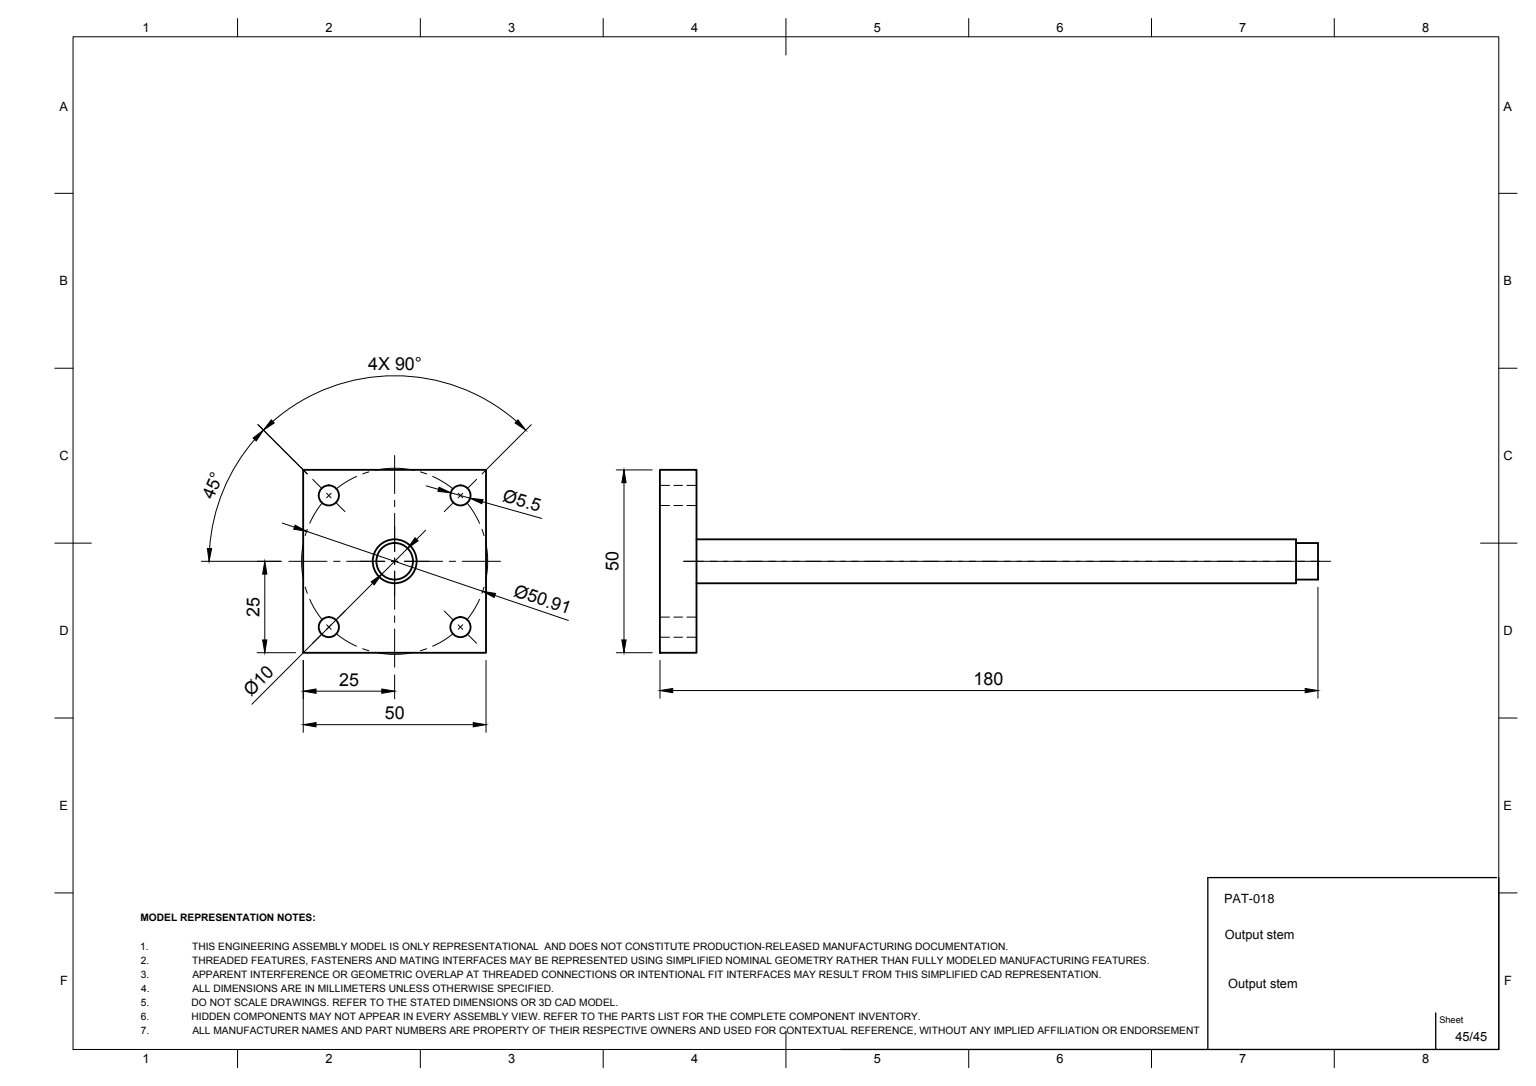
ISO-10303-21;
HEADER;
/* Generated by software containing ST-Developer
 * from STEP Tools, Inc. (www.steptools.com) 
 */

FILE_DESCRIPTION(
/* description */ ('Cam-driven reciprocating slide'),
/* implementation_level */ '2;1');

FILE_NAME(
/* name */ 'Output stem.step',
/* time_stamp */ '2026-10-28T03:25:20-07:00',
/* author */ (''),
/* organization */ (''),
/* preprocessor_version */ 'ST-DEVELOPER v20.2',
/* originating_system */ 'Autodesk Translation Framework v15.17.0.0',
/* authorisation */ '');

FILE_SCHEMA (('AUTOMOTIVE_DESIGN { 1 0 10303 214 3 1 1 }'));
ENDSEC;

DATA;
#10=MECHANICAL_DESIGN_GEOMETRIC_PRESENTATION_REPRESENTATION('',(#464),#13277);
#383=SHAPE_REPRESENTATION_RELATIONSHIP('SRR','None',#13480,#420);
#420=ADVANCED_BREP_SHAPE_REPRESENTATION('',(#505),#13275);
#464=STYLED_ITEM('',(#13706),#505);
#505=MANIFOLD_SOLID_BREP('Body1',#6443);
#669=FACE_BOUND('',#1808,.T.);
#670=FACE_BOUND('',#1809,.T.);
#671=FACE_BOUND('',#1810,.T.);
#672=FACE_BOUND('',#1811,.T.);
#673=FACE_BOUND('',#1812,.T.);
#674=FACE_BOUND('',#1818,.T.);
#675=FACE_BOUND('',#1819,.T.);
#676=FACE_BOUND('',#1820,.T.);
#677=FACE_BOUND('',#1821,.T.);
#678=FACE_BOUND('',#1826,.T.);
#891=PLANE('',#7640);
#892=PLANE('',#7642);
#893=PLANE('',#7643);
#894=PLANE('',#7644);
#895=PLANE('',#7645);
#896=PLANE('',#7646);
#897=PLANE('',#7650);
#898=PLANE('',#7653);
#1262=FACE_OUTER_BOUND('',#1803,.T.);
#1263=FACE_OUTER_BOUND('',#1804,.T.);
#1264=FACE_OUTER_BOUND('',#1805,.T.);
#1265=FACE_OUTER_BOUND('',#1806,.T.);
#1266=FACE_OUTER_BOUND('',#1807,.T.);
#1267=FACE_OUTER_BOUND('',#1813,.T.);
#1268=FACE_OUTER_BOUND('',#1814,.T.);
#1269=FACE_OUTER_BOUND('',#1815,.T.);
#1270=FACE_OUTER_BOUND('',#1816,.T.);
#1271=FACE_OUTER_BOUND('',#1817,.T.);
#1272=FACE_OUTER_BOUND('',#1822,.T.);
#1273=FACE_OUTER_BOUND('',#1823,.T.);
#1274=FACE_OUTER_BOUND('',#1824,.T.);
#1275=FACE_OUTER_BOUND('',#1825,.T.);
#1803=EDGE_LOOP('',(#5820,#5821,#5822,#5823));
#1804=EDGE_LOOP('',(#5824,#5825,#5826,#5827));
#1805=EDGE_LOOP('',(#5828,#5829,#5830,#5831));
#1806=EDGE_LOOP('',(#5832,#5833,#5834,#5835));
#1807=EDGE_LOOP('',(#5836,#5837,#5838,#5839));
#1808=EDGE_LOOP('',(#5840));
#1809=EDGE_LOOP('',(#5841));
#1810=EDGE_LOOP('',(#5842));
#1811=EDGE_LOOP('',(#5843));
#1812=EDGE_LOOP('',(#5844));
#1813=EDGE_LOOP('',(#5845,#5846,#5847,#5848));
#1814=EDGE_LOOP('',(#5849,#5850,#5851,#5852));
#1815=EDGE_LOOP('',(#5853,#5854,#5855,#5856));
#1816=EDGE_LOOP('',(#5857,#5858,#5859,#5860));
#1817=EDGE_LOOP('',(#5861,#5862,#5863,#5864));
#1818=EDGE_LOOP('',(#5865));
#1819=EDGE_LOOP('',(#5866));
#1820=EDGE_LOOP('',(#5867));
#1821=EDGE_LOOP('',(#5868));
#1822=EDGE_LOOP('',(#5869,#5870,#5871,#5872));
#1823=EDGE_LOOP('',(#5873));
#1824=EDGE_LOOP('',(#5874,#5875,#5876,#5877));
#1825=EDGE_LOOP('',(#5878));
#1826=EDGE_LOOP('',(#5879));
#2252=LINE('',#13109,#2691);
#2253=LINE('',#13115,#2692);
#2254=LINE('',#13121,#2693);
#2255=LINE('',#13127,#2694);
#2256=LINE('',#13132,#2695);
#2257=LINE('',#13134,#2696);
#2258=LINE('',#13136,#2697);
#2259=LINE('',#13137,#2698);
#2260=LINE('',#13142,#2699);
#2261=LINE('',#13144,#2700);
#2262=LINE('',#13145,#2701);
#2263=LINE('',#13148,#2702);
#2264=LINE('',#13149,#2703);
#2265=LINE('',#13152,#2704);
#2266=LINE('',#13153,#2705);
#2267=LINE('',#13155,#2706);
#2268=LINE('',#13161,#2707);
#2269=LINE('',#13166,#2708);
#2691=VECTOR('',#9642,0.275);
#2692=VECTOR('',#9649,0.275);
#2693=VECTOR('',#9656,0.275);
#2694=VECTOR('',#9663,0.275);
#2695=VECTOR('',#9668,1.);
#2696=VECTOR('',#9669,1.);
#2697=VECTOR('',#9670,1.);
#2698=VECTOR('',#9671,1.);
#2699=VECTOR('',#9676,1.);
#2700=VECTOR('',#9677,1.);
#2701=VECTOR('',#9678,1.);
#2702=VECTOR('',#9681,1.);
#2703=VECTOR('',#9682,1.);
#2704=VECTOR('',#9685,1.);
#2705=VECTOR('',#9686,1.);
#2706=VECTOR('',#9689,1.);
#2707=VECTOR('',#9696,0.5);
#2708=VECTOR('',#9703,0.6);
#3019=CIRCLE('',#7629,0.275);
#3020=CIRCLE('',#7630,0.275);
#3021=CIRCLE('',#7632,0.275);
#3022=CIRCLE('',#7633,0.275);
#3023=CIRCLE('',#7635,0.275);
#3024=CIRCLE('',#7636,0.275);
#3025=CIRCLE('',#7638,0.275);
#3026=CIRCLE('',#7639,0.275);
#3027=CIRCLE('',#7641,0.6);
#3028=CIRCLE('',#7648,0.5);
#3029=CIRCLE('',#7649,0.5);
#3030=CIRCLE('',#7652,0.6);
#3534=VERTEX_POINT('',#13106);
#3535=VERTEX_POINT('',#13108);
#3536=VERTEX_POINT('',#13112);
#3537=VERTEX_POINT('',#13114);
#3538=VERTEX_POINT('',#13118);
#3539=VERTEX_POINT('',#13120);
#3540=VERTEX_POINT('',#13124);
#3541=VERTEX_POINT('',#13126);
#3542=VERTEX_POINT('',#13130);
#3543=VERTEX_POINT('',#13131);
#3544=VERTEX_POINT('',#13133);
#3545=VERTEX_POINT('',#13135);
#3546=VERTEX_POINT('',#13138);
#3547=VERTEX_POINT('',#13141);
#3548=VERTEX_POINT('',#13143);
#3549=VERTEX_POINT('',#13147);
#3550=VERTEX_POINT('',#13151);
#3551=VERTEX_POINT('',#13158);
#3552=VERTEX_POINT('',#13160);
#3553=VERTEX_POINT('',#13165);
#4300=EDGE_CURVE('',#3534,#3534,#3019,.T.);
#4301=EDGE_CURVE('',#3534,#3535,#2252,.T.);
#4302=EDGE_CURVE('',#3535,#3535,#3020,.T.);
#4303=EDGE_CURVE('',#3536,#3536,#3021,.T.);
#4304=EDGE_CURVE('',#3536,#3537,#2253,.T.);
#4305=EDGE_CURVE('',#3537,#3537,#3022,.T.);
#4306=EDGE_CURVE('',#3538,#3538,#3023,.T.);
#4307=EDGE_CURVE('',#3538,#3539,#2254,.T.);
#4308=EDGE_CURVE('',#3539,#3539,#3024,.T.);
#4309=EDGE_CURVE('',#3540,#3540,#3025,.T.);
#4310=EDGE_CURVE('',#3540,#3541,#2255,.T.);
#4311=EDGE_CURVE('',#3541,#3541,#3026,.T.);
#4312=EDGE_CURVE('',#3542,#3543,#2256,.T.);
#4313=EDGE_CURVE('',#3544,#3542,#2257,.T.);
#4314=EDGE_CURVE('',#3545,#3544,#2258,.T.);
#4315=EDGE_CURVE('',#3543,#3545,#2259,.T.);
#4316=EDGE_CURVE('',#3546,#3546,#3027,.T.);
#4317=EDGE_CURVE('',#3542,#3547,#2260,.T.);
#4318=EDGE_CURVE('',#3548,#3547,#2261,.T.);
#4319=EDGE_CURVE('',#3544,#3548,#2262,.T.);
#4320=EDGE_CURVE('',#3549,#3548,#2263,.T.);
#4321=EDGE_CURVE('',#3545,#3549,#2264,.T.);
#4322=EDGE_CURVE('',#3550,#3549,#2265,.T.);
#4323=EDGE_CURVE('',#3543,#3550,#2266,.T.);
#4324=EDGE_CURVE('',#3547,#3550,#2267,.T.);
#4325=EDGE_CURVE('',#3551,#3551,#3028,.T.);
#4326=EDGE_CURVE('',#3551,#3552,#2268,.T.);
#4327=EDGE_CURVE('',#3552,#3552,#3029,.T.);
#4328=EDGE_CURVE('',#3546,#3553,#2269,.T.);
#4329=EDGE_CURVE('',#3553,#3553,#3030,.T.);
#5820=ORIENTED_EDGE('',*,*,#4300,.F.);
#5821=ORIENTED_EDGE('',*,*,#4301,.T.);
#5822=ORIENTED_EDGE('',*,*,#4302,.F.);
#5823=ORIENTED_EDGE('',*,*,#4301,.F.);
#5824=ORIENTED_EDGE('',*,*,#4303,.F.);
#5825=ORIENTED_EDGE('',*,*,#4304,.T.);
#5826=ORIENTED_EDGE('',*,*,#4305,.F.);
#5827=ORIENTED_EDGE('',*,*,#4304,.F.);
#5828=ORIENTED_EDGE('',*,*,#4306,.F.);
#5829=ORIENTED_EDGE('',*,*,#4307,.T.);
#5830=ORIENTED_EDGE('',*,*,#4308,.F.);
#5831=ORIENTED_EDGE('',*,*,#4307,.F.);
#5832=ORIENTED_EDGE('',*,*,#4309,.F.);
#5833=ORIENTED_EDGE('',*,*,#4310,.T.);
#5834=ORIENTED_EDGE('',*,*,#4311,.F.);
#5835=ORIENTED_EDGE('',*,*,#4310,.F.);
#5836=ORIENTED_EDGE('',*,*,#4312,.F.);
#5837=ORIENTED_EDGE('',*,*,#4313,.F.);
#5838=ORIENTED_EDGE('',*,*,#4314,.F.);
#5839=ORIENTED_EDGE('',*,*,#4315,.F.);
#5840=ORIENTED_EDGE('',*,*,#4316,.T.);
#5841=ORIENTED_EDGE('',*,*,#4309,.T.);
#5842=ORIENTED_EDGE('',*,*,#4306,.T.);
#5843=ORIENTED_EDGE('',*,*,#4303,.T.);
#5844=ORIENTED_EDGE('',*,*,#4300,.T.);
#5845=ORIENTED_EDGE('',*,*,#4313,.T.);
#5846=ORIENTED_EDGE('',*,*,#4317,.T.);
#5847=ORIENTED_EDGE('',*,*,#4318,.F.);
#5848=ORIENTED_EDGE('',*,*,#4319,.F.);
#5849=ORIENTED_EDGE('',*,*,#4314,.T.);
#5850=ORIENTED_EDGE('',*,*,#4319,.T.);
#5851=ORIENTED_EDGE('',*,*,#4320,.F.);
#5852=ORIENTED_EDGE('',*,*,#4321,.F.);
#5853=ORIENTED_EDGE('',*,*,#4315,.T.);
#5854=ORIENTED_EDGE('',*,*,#4321,.T.);
#5855=ORIENTED_EDGE('',*,*,#4322,.F.);
#5856=ORIENTED_EDGE('',*,*,#4323,.F.);
#5857=ORIENTED_EDGE('',*,*,#4312,.T.);
#5858=ORIENTED_EDGE('',*,*,#4323,.T.);
#5859=ORIENTED_EDGE('',*,*,#4324,.F.);
#5860=ORIENTED_EDGE('',*,*,#4317,.F.);
#5861=ORIENTED_EDGE('',*,*,#4324,.T.);
#5862=ORIENTED_EDGE('',*,*,#4322,.T.);
#5863=ORIENTED_EDGE('',*,*,#4320,.T.);
#5864=ORIENTED_EDGE('',*,*,#4318,.T.);
#5865=ORIENTED_EDGE('',*,*,#4302,.T.);
#5866=ORIENTED_EDGE('',*,*,#4305,.T.);
#5867=ORIENTED_EDGE('',*,*,#4308,.T.);
#5868=ORIENTED_EDGE('',*,*,#4311,.T.);
#5869=ORIENTED_EDGE('',*,*,#4325,.F.);
#5870=ORIENTED_EDGE('',*,*,#4326,.T.);
#5871=ORIENTED_EDGE('',*,*,#4327,.T.);
#5872=ORIENTED_EDGE('',*,*,#4326,.F.);
#5873=ORIENTED_EDGE('',*,*,#4327,.F.);
#5874=ORIENTED_EDGE('',*,*,#4316,.F.);
#5875=ORIENTED_EDGE('',*,*,#4328,.T.);
#5876=ORIENTED_EDGE('',*,*,#4329,.T.);
#5877=ORIENTED_EDGE('',*,*,#4328,.F.);
#5878=ORIENTED_EDGE('',*,*,#4329,.F.);
#5879=ORIENTED_EDGE('',*,*,#4325,.T.);
#6011=CYLINDRICAL_SURFACE('',#7628,0.275);
#6012=CYLINDRICAL_SURFACE('',#7631,0.275);
#6013=CYLINDRICAL_SURFACE('',#7634,0.275);
#6014=CYLINDRICAL_SURFACE('',#7637,0.275);
#6015=CYLINDRICAL_SURFACE('',#7647,0.5);
#6016=CYLINDRICAL_SURFACE('',#7651,0.6);
#6380=ADVANCED_FACE('',(#1262),#6011,.F.);
#6381=ADVANCED_FACE('',(#1263),#6012,.F.);
#6382=ADVANCED_FACE('',(#1264),#6013,.F.);
#6383=ADVANCED_FACE('',(#1265),#6014,.F.);
#6384=ADVANCED_FACE('',(#1266,#669,#670,#671,#672,#673),#891,.F.);
#6385=ADVANCED_FACE('',(#1267),#892,.T.);
#6386=ADVANCED_FACE('',(#1268),#893,.T.);
#6387=ADVANCED_FACE('',(#1269),#894,.T.);
#6388=ADVANCED_FACE('',(#1270),#895,.T.);
#6389=ADVANCED_FACE('',(#1271,#674,#675,#676,#677),#896,.T.);
#6390=ADVANCED_FACE('',(#1272),#6015,.T.);
#6391=ADVANCED_FACE('',(#1273),#897,.F.);
#6392=ADVANCED_FACE('',(#1274),#6016,.T.);
#6393=ADVANCED_FACE('',(#1275,#678),#898,.F.);
#6443=CLOSED_SHELL('',(#6380,#6381,#6382,#6383,#6384,#6385,#6386,#6387,
#6388,#6389,#6390,#6391,#6392,#6393));
#7627=AXIS2_PLACEMENT_3D('',#13104,#9636,#9637);
#7628=AXIS2_PLACEMENT_3D('',#13105,#9638,#9639);
#7629=AXIS2_PLACEMENT_3D('',#13107,#9640,#9641);
#7630=AXIS2_PLACEMENT_3D('',#13110,#9643,#9644);
#7631=AXIS2_PLACEMENT_3D('',#13111,#9645,#9646);
#7632=AXIS2_PLACEMENT_3D('',#13113,#9647,#9648);
#7633=AXIS2_PLACEMENT_3D('',#13116,#9650,#9651);
#7634=AXIS2_PLACEMENT_3D('',#13117,#9652,#9653);
#7635=AXIS2_PLACEMENT_3D('',#13119,#9654,#9655);
#7636=AXIS2_PLACEMENT_3D('',#13122,#9657,#9658);
#7637=AXIS2_PLACEMENT_3D('',#13123,#9659,#9660);
#7638=AXIS2_PLACEMENT_3D('',#13125,#9661,#9662);
#7639=AXIS2_PLACEMENT_3D('',#13128,#9664,#9665);
#7640=AXIS2_PLACEMENT_3D('',#13129,#9666,#9667);
#7641=AXIS2_PLACEMENT_3D('',#13139,#9672,#9673);
#7642=AXIS2_PLACEMENT_3D('',#13140,#9674,#9675);
#7643=AXIS2_PLACEMENT_3D('',#13146,#9679,#9680);
#7644=AXIS2_PLACEMENT_3D('',#13150,#9683,#9684);
#7645=AXIS2_PLACEMENT_3D('',#13154,#9687,#9688);
#7646=AXIS2_PLACEMENT_3D('',#13156,#9690,#9691);
#7647=AXIS2_PLACEMENT_3D('',#13157,#9692,#9693);
#7648=AXIS2_PLACEMENT_3D('',#13159,#9694,#9695);
#7649=AXIS2_PLACEMENT_3D('',#13162,#9697,#9698);
#7650=AXIS2_PLACEMENT_3D('',#13163,#9699,#9700);
#7651=AXIS2_PLACEMENT_3D('',#13164,#9701,#9702);
#7652=AXIS2_PLACEMENT_3D('',#13167,#9704,#9705);
#7653=AXIS2_PLACEMENT_3D('',#13168,#9706,#9707);
#9636=DIRECTION('axis',(0.,0.,1.));
#9637=DIRECTION('refdir',(1.,0.,0.));
#9638=DIRECTION('center_axis',(0.,0.,1.));
#9639=DIRECTION('ref_axis',(1.,0.,0.));
#9640=DIRECTION('center_axis',(0.,0.,1.));
#9641=DIRECTION('ref_axis',(1.,0.,0.));
#9642=DIRECTION('',(0.,0.,1.));
#9643=DIRECTION('center_axis',(0.,0.,-1.));
#9644=DIRECTION('ref_axis',(1.,0.,0.));
#9645=DIRECTION('center_axis',(0.,0.,1.));
#9646=DIRECTION('ref_axis',(1.,0.,0.));
#9647=DIRECTION('center_axis',(0.,0.,1.));
#9648=DIRECTION('ref_axis',(1.,0.,0.));
#9649=DIRECTION('',(0.,0.,1.));
#9650=DIRECTION('center_axis',(0.,0.,-1.));
#9651=DIRECTION('ref_axis',(1.,0.,0.));
#9652=DIRECTION('center_axis',(0.,0.,1.));
#9653=DIRECTION('ref_axis',(1.,0.,0.));
#9654=DIRECTION('center_axis',(0.,0.,1.));
#9655=DIRECTION('ref_axis',(1.,0.,0.));
#9656=DIRECTION('',(0.,0.,1.));
#9657=DIRECTION('center_axis',(0.,0.,-1.));
#9658=DIRECTION('ref_axis',(1.,0.,0.));
#9659=DIRECTION('center_axis',(0.,0.,1.));
#9660=DIRECTION('ref_axis',(1.,0.,0.));
#9661=DIRECTION('center_axis',(0.,0.,1.));
#9662=DIRECTION('ref_axis',(1.,0.,0.));
#9663=DIRECTION('',(0.,0.,1.));
#9664=DIRECTION('center_axis',(0.,0.,-1.));
#9665=DIRECTION('ref_axis',(1.,0.,0.));
#9666=DIRECTION('center_axis',(0.,0.,1.));
#9667=DIRECTION('ref_axis',(1.,0.,0.));
#9668=DIRECTION('',(0.,-1.,0.));
#9669=DIRECTION('',(-1.,0.,0.));
#9670=DIRECTION('',(0.,1.,0.));
#9671=DIRECTION('',(1.,0.,0.));
#9672=DIRECTION('center_axis',(0.,0.,1.));
#9673=DIRECTION('ref_axis',(1.,0.,0.));
#9674=DIRECTION('center_axis',(0.,1.,0.));
#9675=DIRECTION('ref_axis',(-1.,0.,0.));
#9676=DIRECTION('',(0.,0.,1.));
#9677=DIRECTION('',(-1.,0.,0.));
#9678=DIRECTION('',(0.,0.,1.));
#9679=DIRECTION('center_axis',(1.,0.,0.));
#9680=DIRECTION('ref_axis',(0.,1.,0.));
#9681=DIRECTION('',(0.,1.,0.));
#9682=DIRECTION('',(0.,0.,1.));
#9683=DIRECTION('center_axis',(0.,-1.,0.));
#9684=DIRECTION('ref_axis',(1.,0.,0.));
#9685=DIRECTION('',(1.,0.,0.));
#9686=DIRECTION('',(0.,0.,1.));
#9687=DIRECTION('center_axis',(-1.,0.,0.));
#9688=DIRECTION('ref_axis',(0.,-1.,0.));
#9689=DIRECTION('',(0.,-1.,0.));
#9690=DIRECTION('center_axis',(0.,0.,1.));
#9691=DIRECTION('ref_axis',(1.,0.,0.));
#9692=DIRECTION('center_axis',(0.,0.,1.));
#9693=DIRECTION('ref_axis',(1.,0.,0.));
#9694=DIRECTION('center_axis',(0.,0.,1.));
#9695=DIRECTION('ref_axis',(1.,0.,0.));
#9696=DIRECTION('',(0.,0.,-1.));
#9697=DIRECTION('center_axis',(0.,0.,1.));
#9698=DIRECTION('ref_axis',(1.,0.,0.));
#9699=DIRECTION('center_axis',(0.,0.,1.));
#9700=DIRECTION('ref_axis',(1.,0.,0.));
#9701=DIRECTION('center_axis',(0.,0.,1.));
#9702=DIRECTION('ref_axis',(1.,0.,0.));
#9703=DIRECTION('',(0.,0.,-1.));
#9704=DIRECTION('center_axis',(0.,0.,1.));
#9705=DIRECTION('ref_axis',(1.,0.,0.));
#9706=DIRECTION('center_axis',(0.,0.,1.));
#9707=DIRECTION('ref_axis',(1.,0.,0.));
#13104=CARTESIAN_POINT('',(0.,0.,0.));
#13105=CARTESIAN_POINT('Origin',(1.8,-1.8,23.9));
#13106=CARTESIAN_POINT('',(1.525,-1.8,24.));
#13107=CARTESIAN_POINT('Origin',(1.8,-1.8,24.));
#13108=CARTESIAN_POINT('',(1.525,-1.8,25.));
#13109=CARTESIAN_POINT('',(1.525,-1.8,23.9));
#13110=CARTESIAN_POINT('Origin',(1.8,-1.8,25.));
#13111=CARTESIAN_POINT('Origin',(-1.8,1.8,23.9));
#13112=CARTESIAN_POINT('',(-2.075,1.8,24.));
#13113=CARTESIAN_POINT('Origin',(-1.8,1.8,24.));
#13114=CARTESIAN_POINT('',(-2.075,1.8,25.));
#13115=CARTESIAN_POINT('',(-2.075,1.8,23.9));
#13116=CARTESIAN_POINT('Origin',(-1.8,1.8,25.));
#13117=CARTESIAN_POINT('Origin',(-1.8,-1.8,23.9));
#13118=CARTESIAN_POINT('',(-2.075,-1.8,24.));
#13119=CARTESIAN_POINT('Origin',(-1.8,-1.8,24.));
#13120=CARTESIAN_POINT('',(-2.075,-1.8,25.));
#13121=CARTESIAN_POINT('',(-2.075,-1.8,23.9));
#13122=CARTESIAN_POINT('Origin',(-1.8,-1.8,25.));
#13123=CARTESIAN_POINT('Origin',(1.8,1.8,23.9));
#13124=CARTESIAN_POINT('',(1.525,1.8,24.));
#13125=CARTESIAN_POINT('Origin',(1.8,1.8,24.));
#13126=CARTESIAN_POINT('',(1.525,1.8,25.));
#13127=CARTESIAN_POINT('',(1.525,1.8,23.9));
#13128=CARTESIAN_POINT('Origin',(1.8,1.8,25.));
#13129=CARTESIAN_POINT('Origin',(0.,0.,24.));
#13130=CARTESIAN_POINT('',(-2.5,2.5,24.));
#13131=CARTESIAN_POINT('',(-2.5,-2.5,24.));
#13132=CARTESIAN_POINT('',(-2.5,2.5,24.));
#13133=CARTESIAN_POINT('',(2.5,2.5,24.));
#13134=CARTESIAN_POINT('',(2.5,2.5,24.));
#13135=CARTESIAN_POINT('',(2.5,-2.5,24.));
#13136=CARTESIAN_POINT('',(2.5,-2.5,24.));
#13137=CARTESIAN_POINT('',(-2.5,-2.5,24.));
#13138=CARTESIAN_POINT('',(-0.6,-7.34788079488412E-17,24.));
#13139=CARTESIAN_POINT('Origin',(0.,0.,24.));
#13140=CARTESIAN_POINT('Origin',(2.5,2.5,24.));
#13141=CARTESIAN_POINT('',(-2.5,2.5,25.));
#13142=CARTESIAN_POINT('',(-2.5,2.5,24.));
#13143=CARTESIAN_POINT('',(2.5,2.5,25.));
#13144=CARTESIAN_POINT('',(2.5,2.5,25.));
#13145=CARTESIAN_POINT('',(2.5,2.5,24.));
#13146=CARTESIAN_POINT('Origin',(2.5,-2.5,24.));
#13147=CARTESIAN_POINT('',(2.5,-2.5,25.));
#13148=CARTESIAN_POINT('',(2.5,-2.5,25.));
#13149=CARTESIAN_POINT('',(2.5,-2.5,24.));
#13150=CARTESIAN_POINT('Origin',(-2.5,-2.5,24.));
#13151=CARTESIAN_POINT('',(-2.5,-2.5,25.));
#13152=CARTESIAN_POINT('',(-2.5,-2.5,25.));
#13153=CARTESIAN_POINT('',(-2.5,-2.5,24.));
#13154=CARTESIAN_POINT('Origin',(-2.5,2.5,24.));
#13155=CARTESIAN_POINT('',(-2.5,2.5,25.));
#13156=CARTESIAN_POINT('Origin',(0.,0.,25.));
#13157=CARTESIAN_POINT('Origin',(0.,0.,7.));
#13158=CARTESIAN_POINT('',(-0.5,-6.12323399573677E-17,7.6));
#13159=CARTESIAN_POINT('Origin',(0.,0.,7.6));
#13160=CARTESIAN_POINT('',(-0.5,-6.12323399573677E-17,7.));
#13161=CARTESIAN_POINT('',(-0.5,-6.12323399573677E-17,7.));
#13162=CARTESIAN_POINT('Origin',(0.,0.,7.));
#13163=CARTESIAN_POINT('Origin',(0.,0.,7.));
#13164=CARTESIAN_POINT('Origin',(0.,0.,7.6));
#13165=CARTESIAN_POINT('',(-0.6,-7.34788079488412E-17,7.6));
#13166=CARTESIAN_POINT('',(-0.6,-7.34788079488412E-17,7.6));
#13167=CARTESIAN_POINT('Origin',(0.,0.,7.6));
#13168=CARTESIAN_POINT('Origin',(0.,0.,7.6));
#13231=UNCERTAINTY_MEASURE_WITH_UNIT(LENGTH_MEASURE(0.001),#13278,
'DISTANCE_ACCURACY_VALUE',
'Maximum model space distance between geometric entities at asserted c
onnectivities');
#13233=UNCERTAINTY_MEASURE_WITH_UNIT(LENGTH_MEASURE(0.001),#13278,
'DISTANCE_ACCURACY_VALUE',
'Maximum model space distance between geometric entities at asserted c
onnectivities');
#13275=(
GEOMETRIC_REPRESENTATION_CONTEXT(3)
GLOBAL_UNCERTAINTY_ASSIGNED_CONTEXT((#13231))
GLOBAL_UNIT_ASSIGNED_CONTEXT((#13278,#13280,#13281))
REPRESENTATION_CONTEXT('','3D')
);
#13277=(
GEOMETRIC_REPRESENTATION_CONTEXT(3)
GLOBAL_UNCERTAINTY_ASSIGNED_CONTEXT((#13233))
GLOBAL_UNIT_ASSIGNED_CONTEXT((#13278,#13280,#13281))
REPRESENTATION_CONTEXT('','3D')
);
#13278=(
LENGTH_UNIT()
NAMED_UNIT(*)
SI_UNIT(.CENTI.,.METRE.)
);
#13280=(
NAMED_UNIT(*)
PLANE_ANGLE_UNIT()
SI_UNIT($,.RADIAN.)
);
#13281=(
NAMED_UNIT(*)
SI_UNIT($,.STERADIAN.)
SOLID_ANGLE_UNIT()
);
#13323=SHAPE_DEFINITION_REPRESENTATION(#13431,#13480);
#13431=PRODUCT_DEFINITION_SHAPE('',$,#13524);
#13480=SHAPE_REPRESENTATION('',(#7627),#13275);
#13482=PRODUCT_DEFINITION_CONTEXT('part definition',#13613,'design');
#13524=PRODUCT_DEFINITION('Output stem','Output stem',#13567,#13482);
#13567=PRODUCT_DEFINITION_FORMATION('',$,#13656);
#13613=APPLICATION_CONTEXT(
'Core Data for Automotive Mechanical Design Process');
#13614=PRODUCT_CONTEXT('part definition',#13613,'mechanical');
#13656=PRODUCT('Output stem','Output stem','Output stem',(#13614));
#13700=COLOUR_RGB('Light Blue',0.38,0.62,0.78);
#13701=FILL_AREA_STYLE_COLOUR('',#13700);
#13702=FILL_AREA_STYLE('',(#13701));
#13703=SURFACE_STYLE_FILL_AREA(#13702);
#13704=SURFACE_SIDE_STYLE('',(#13703));
#13705=SURFACE_STYLE_USAGE(.BOTH.,#13704);
#13706=PRESENTATION_STYLE_ASSIGNMENT((#13705));
ENDSEC;
END-ISO-10303-21;
